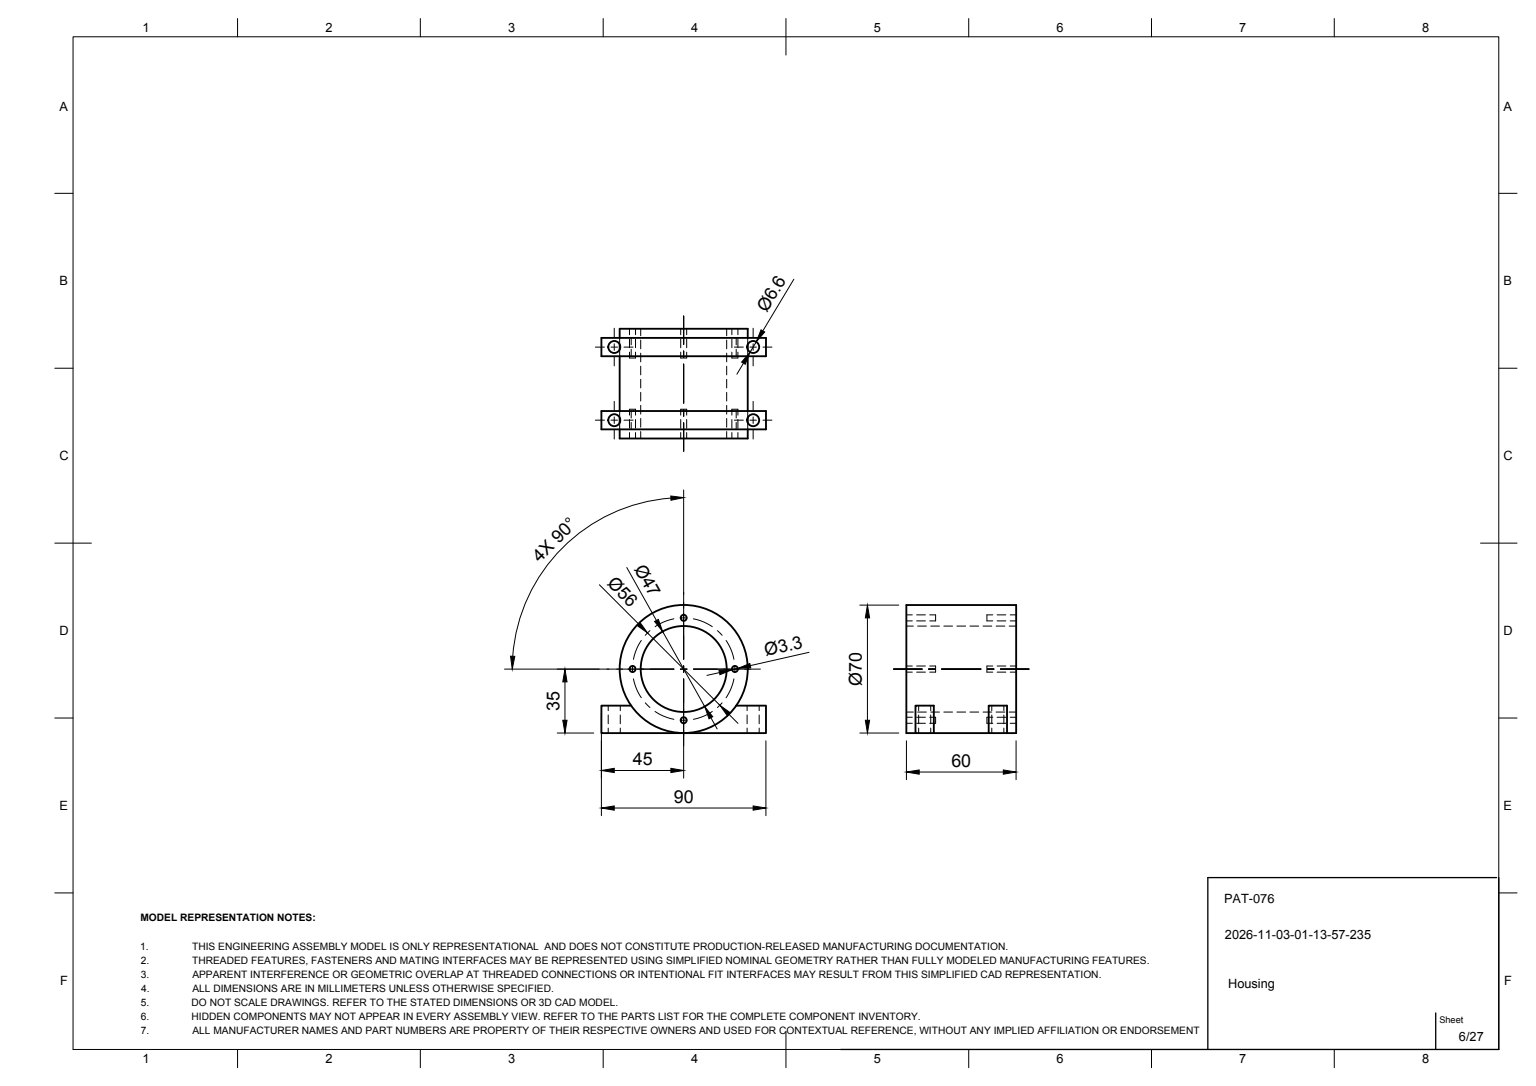
ISO-10303-21;
HEADER;
/* Generated by software containing ST-Developer
 * from STEP Tools, Inc. (www.steptools.com) 
 */

FILE_DESCRIPTION(
/* description */ ('Overhung pulley bearing cartridge'),
/* implementation_level */ '2;1');

FILE_NAME(
/* name */ 'Housing.step',
/* time_stamp */ '2026-10-28T03:22:33-07:00',
/* author */ (''),
/* organization */ (''),
/* preprocessor_version */ 'ST-DEVELOPER v20.2',
/* originating_system */ 'Autodesk Translation Framework v15.17.0.0',
/* authorisation */ '');

FILE_SCHEMA (('AUTOMOTIVE_DESIGN { 1 0 10303 214 3 1 1 }'));
ENDSEC;

DATA;
#10=MECHANICAL_DESIGN_GEOMETRIC_PRESENTATION_REPRESENTATION('',(#284),#10963);
#240=SHAPE_REPRESENTATION_RELATIONSHIP('SRR','None',#11060,#262);
#262=ADVANCED_BREP_SHAPE_REPRESENTATION('',(#314),#10940);
#284=STYLED_ITEM('',(#11232),#314);
#314=MANIFOLD_SOLID_BREP('Body1',#5651);
#349=FACE_BOUND('',#949,.T.);
#350=FACE_BOUND('',#951,.T.);
#351=FACE_BOUND('',#954,.T.);
#352=FACE_BOUND('',#955,.T.);
#353=FACE_BOUND('',#962,.T.);
#354=FACE_BOUND('',#964,.T.);
#355=FACE_BOUND('',#967,.T.);
#356=FACE_BOUND('',#968,.T.);
#357=FACE_BOUND('',#972,.T.);
#358=FACE_BOUND('',#973,.T.);
#359=FACE_BOUND('',#975,.T.);
#360=FACE_BOUND('',#976,.T.);
#361=FACE_BOUND('',#977,.T.);
#362=FACE_BOUND('',#978,.T.);
#363=FACE_BOUND('',#979,.T.);
#364=FACE_BOUND('',#981,.T.);
#365=FACE_BOUND('',#982,.T.);
#366=FACE_BOUND('',#983,.T.);
#367=FACE_BOUND('',#984,.T.);
#368=FACE_BOUND('',#985,.T.);
#440=PLANE('',#5950);
#441=PLANE('',#5954);
#442=PLANE('',#5958);
#443=PLANE('',#5962);
#444=PLANE('',#5966);
#445=PLANE('',#5970);
#446=PLANE('',#5974);
#447=PLANE('',#5978);
#448=PLANE('',#5991);
#449=PLANE('',#5993);
#450=PLANE('',#5995);
#451=PLANE('',#5997);
#452=PLANE('',#5999);
#453=PLANE('',#6000);
#454=PLANE('',#6001);
#455=PLANE('',#6002);
#456=PLANE('',#6003);
#457=PLANE('',#6004);
#458=PLANE('',#6006);
#459=PLANE('',#6008);
#460=PLANE('',#6010);
#461=PLANE('',#6012);
#462=PLANE('',#6013);
#463=PLANE('',#6014);
#464=PLANE('',#6015);
#465=PLANE('',#6016);
#466=PLANE('',#6023);
#467=PLANE('',#6024);
#587=FACE_OUTER_BOUND('',#924,.T.);
#588=FACE_OUTER_BOUND('',#925,.T.);
#589=FACE_OUTER_BOUND('',#926,.T.);
#590=FACE_OUTER_BOUND('',#927,.T.);
#591=FACE_OUTER_BOUND('',#928,.T.);
#592=FACE_OUTER_BOUND('',#929,.T.);
#593=FACE_OUTER_BOUND('',#930,.T.);
#594=FACE_OUTER_BOUND('',#931,.T.);
#595=FACE_OUTER_BOUND('',#932,.T.);
#596=FACE_OUTER_BOUND('',#933,.T.);
#597=FACE_OUTER_BOUND('',#934,.T.);
#598=FACE_OUTER_BOUND('',#935,.T.);
#599=FACE_OUTER_BOUND('',#936,.T.);
#600=FACE_OUTER_BOUND('',#937,.T.);
#601=FACE_OUTER_BOUND('',#938,.T.);
#602=FACE_OUTER_BOUND('',#939,.T.);
#603=FACE_OUTER_BOUND('',#940,.T.);
#604=FACE_OUTER_BOUND('',#941,.T.);
#605=FACE_OUTER_BOUND('',#942,.T.);
#606=FACE_OUTER_BOUND('',#943,.T.);
#607=FACE_OUTER_BOUND('',#944,.T.);
#608=FACE_OUTER_BOUND('',#945,.T.);
#609=FACE_OUTER_BOUND('',#946,.T.);
#610=FACE_OUTER_BOUND('',#947,.T.);
#611=FACE_OUTER_BOUND('',#948,.T.);
#612=FACE_OUTER_BOUND('',#950,.T.);
#613=FACE_OUTER_BOUND('',#952,.T.);
#614=FACE_OUTER_BOUND('',#953,.T.);
#615=FACE_OUTER_BOUND('',#956,.T.);
#616=FACE_OUTER_BOUND('',#957,.T.);
#617=FACE_OUTER_BOUND('',#958,.T.);
#618=FACE_OUTER_BOUND('',#959,.T.);
#619=FACE_OUTER_BOUND('',#960,.T.);
#620=FACE_OUTER_BOUND('',#961,.T.);
#621=FACE_OUTER_BOUND('',#963,.T.);
#622=FACE_OUTER_BOUND('',#965,.T.);
#623=FACE_OUTER_BOUND('',#966,.T.);
#624=FACE_OUTER_BOUND('',#969,.T.);
#625=FACE_OUTER_BOUND('',#970,.T.);
#626=FACE_OUTER_BOUND('',#971,.T.);
#627=FACE_OUTER_BOUND('',#974,.T.);
#628=FACE_OUTER_BOUND('',#980,.T.);
#924=EDGE_LOOP('',(#3701,#3702,#3703,#3704));
#925=EDGE_LOOP('',(#3705));
#926=EDGE_LOOP('',(#3706,#3707,#3708,#3709));
#927=EDGE_LOOP('',(#3710));
#928=EDGE_LOOP('',(#3711,#3712,#3713,#3714));
#929=EDGE_LOOP('',(#3715));
#930=EDGE_LOOP('',(#3716,#3717,#3718,#3719));
#931=EDGE_LOOP('',(#3720));
#932=EDGE_LOOP('',(#3721,#3722,#3723,#3724));
#933=EDGE_LOOP('',(#3725));
#934=EDGE_LOOP('',(#3726,#3727,#3728,#3729));
#935=EDGE_LOOP('',(#3730));
#936=EDGE_LOOP('',(#3731,#3732,#3733,#3734));
#937=EDGE_LOOP('',(#3735));
#938=EDGE_LOOP('',(#3736,#3737,#3738,#3739));
#939=EDGE_LOOP('',(#3740));
#940=EDGE_LOOP('',(#3741,#3742,#3743,#3744));
#941=EDGE_LOOP('',(#3745,#3746,#3747,#3748));
#942=EDGE_LOOP('',(#3749,#3750,#3751,#3752));
#943=EDGE_LOOP('',(#3753,#3754,#3755,#3756));
#944=EDGE_LOOP('',(#3757,#3758,#3759,#3760));
#945=EDGE_LOOP('',(#3761,#3762,#3763,#3764));
#946=EDGE_LOOP('',(#3765,#3766,#3767,#3768));
#947=EDGE_LOOP('',(#3769,#3770,#3771,#3772));
#948=EDGE_LOOP('',(#3773,#3774,#3775,#3776));
#949=EDGE_LOOP('',(#3777));
#950=EDGE_LOOP('',(#3778,#3779,#3780,#3781));
#951=EDGE_LOOP('',(#3782));
#952=EDGE_LOOP('',(#3783,#3784,#3785,#3786));
#953=EDGE_LOOP('',(#3787,#3788,#3789,#3790,#3791,#3792));
#954=EDGE_LOOP('',(#3793));
#955=EDGE_LOOP('',(#3794));
#956=EDGE_LOOP('',(#3795,#3796,#3797,#3798));
#957=EDGE_LOOP('',(#3799,#3800,#3801,#3802));
#958=EDGE_LOOP('',(#3803,#3804,#3805,#3806));
#959=EDGE_LOOP('',(#3807,#3808,#3809,#3810));
#960=EDGE_LOOP('',(#3811,#3812,#3813,#3814));
#961=EDGE_LOOP('',(#3815,#3816,#3817,#3818));
#962=EDGE_LOOP('',(#3819));
#963=EDGE_LOOP('',(#3820,#3821,#3822,#3823));
#964=EDGE_LOOP('',(#3824));
#965=EDGE_LOOP('',(#3825,#3826,#3827,#3828));
#966=EDGE_LOOP('',(#3829,#3830,#3831,#3832,#3833,#3834));
#967=EDGE_LOOP('',(#3835));
#968=EDGE_LOOP('',(#3836));
#969=EDGE_LOOP('',(#3837,#3838,#3839,#3840));
#970=EDGE_LOOP('',(#3841,#3842,#3843,#3844));
#971=EDGE_LOOP('',(#3845,#3846,#3847,#3848));
#972=EDGE_LOOP('',(#3849,#3850,#3851,#3852,#3853,#3854));
#973=EDGE_LOOP('',(#3855,#3856,#3857,#3858,#3859,#3860));
#974=EDGE_LOOP('',(#3861));
#975=EDGE_LOOP('',(#3862));
#976=EDGE_LOOP('',(#3863));
#977=EDGE_LOOP('',(#3864));
#978=EDGE_LOOP('',(#3865));
#979=EDGE_LOOP('',(#3866));
#980=EDGE_LOOP('',(#3867));
#981=EDGE_LOOP('',(#3868));
#982=EDGE_LOOP('',(#3869));
#983=EDGE_LOOP('',(#3870));
#984=EDGE_LOOP('',(#3871));
#985=EDGE_LOOP('',(#3872));
#1344=LINE('',#8614,#1686);
#1345=LINE('',#8621,#1687);
#1346=LINE('',#8628,#1688);
#1347=LINE('',#8635,#1689);
#1348=LINE('',#8642,#1690);
#1349=LINE('',#8649,#1691);
#1350=LINE('',#8656,#1692);
#1351=LINE('',#8663,#1693);
#1352=LINE('',#8670,#1694);
#1353=LINE('',#8676,#1695);
#1354=LINE('',#8682,#1696);
#1355=LINE('',#8688,#1697);
#1356=LINE('',#8695,#1698);
#1357=LINE('',#8697,#1699);
#1358=LINE('',#8698,#1700);
#1359=LINE('',#8703,#1701);
#1360=LINE('',#8705,#1702);
#1361=LINE('',#8706,#1703);
#1362=LINE('',#8712,#1704);
#1363=LINE('',#8714,#1705);
#1364=LINE('',#8715,#1706);
#1365=LINE('',#8720,#1707);
#1366=LINE('',#8722,#1708);
#1367=LINE('',#8723,#1709);
#1368=LINE('',#8725,#1710);
#1369=LINE('',#8726,#1711);
#1370=LINE('',#8728,#1712);
#1371=LINE('',#8729,#1713);
#1372=LINE('',#8731,#1714);
#1373=LINE('',#8733,#1715);
#1374=LINE('',#8740,#1716);
#1375=LINE('',#8742,#1717);
#1376=LINE('',#8743,#1718);
#1377=LINE('',#8748,#1719);
#1378=LINE('',#8750,#1720);
#1379=LINE('',#8751,#1721);
#1380=LINE('',#8757,#1722);
#1381=LINE('',#8759,#1723);
#1382=LINE('',#8760,#1724);
#1383=LINE('',#8765,#1725);
#1384=LINE('',#8767,#1726);
#1385=LINE('',#8768,#1727);
#1386=LINE('',#8770,#1728);
#1387=LINE('',#8771,#1729);
#1388=LINE('',#8773,#1730);
#1389=LINE('',#8774,#1731);
#1390=LINE('',#8776,#1732);
#1391=LINE('',#8778,#1733);
#1392=LINE('',#8784,#1734);
#1393=LINE('',#8790,#1735);
#1686=VECTOR('',#6752,0.165);
#1687=VECTOR('',#6761,0.165);
#1688=VECTOR('',#6770,0.165);
#1689=VECTOR('',#6779,0.165);
#1690=VECTOR('',#6788,0.165);
#1691=VECTOR('',#6797,0.165);
#1692=VECTOR('',#6806,0.165);
#1693=VECTOR('',#6815,0.165);
#1694=VECTOR('',#6824,0.33);
#1695=VECTOR('',#6831,0.33);
#1696=VECTOR('',#6838,0.33);
#1697=VECTOR('',#6845,0.33);
#1698=VECTOR('',#6852,1.);
#1699=VECTOR('',#6853,1.);
#1700=VECTOR('',#6854,1.);
#1701=VECTOR('',#6859,1.);
#1702=VECTOR('',#6860,1.);
#1703=VECTOR('',#6861,1.);
#1704=VECTOR('',#6866,1.);
#1705=VECTOR('',#6867,1.);
#1706=VECTOR('',#6868,1.);
#1707=VECTOR('',#6873,1.);
#1708=VECTOR('',#6874,1.);
#1709=VECTOR('',#6875,1.);
#1710=VECTOR('',#6878,1.);
#1711=VECTOR('',#6879,1.);
#1712=VECTOR('',#6882,1.);
#1713=VECTOR('',#6883,1.);
#1714=VECTOR('',#6886,1.);
#1715=VECTOR('',#6889,1.);
#1716=VECTOR('',#6896,1.);
#1717=VECTOR('',#6897,1.);
#1718=VECTOR('',#6898,1.);
#1719=VECTOR('',#6903,1.);
#1720=VECTOR('',#6904,1.);
#1721=VECTOR('',#6905,1.);
#1722=VECTOR('',#6910,1.);
#1723=VECTOR('',#6911,1.);
#1724=VECTOR('',#6912,1.);
#1725=VECTOR('',#6917,1.);
#1726=VECTOR('',#6918,1.);
#1727=VECTOR('',#6919,1.);
#1728=VECTOR('',#6922,1.);
#1729=VECTOR('',#6923,1.);
#1730=VECTOR('',#6926,1.);
#1731=VECTOR('',#6927,1.);
#1732=VECTOR('',#6930,1.);
#1733=VECTOR('',#6933,1.);
#1734=VECTOR('',#6940,2.35);
#1735=VECTOR('',#6947,3.5);
#2020=CIRCLE('',#5948,0.165);
#2021=CIRCLE('',#5949,0.165);
#2022=CIRCLE('',#5952,0.165);
#2023=CIRCLE('',#5953,0.165);
#2024=CIRCLE('',#5956,0.165);
#2025=CIRCLE('',#5957,0.165);
#2026=CIRCLE('',#5960,0.165);
#2027=CIRCLE('',#5961,0.165);
#2028=CIRCLE('',#5964,0.165);
#2029=CIRCLE('',#5965,0.165);
#2030=CIRCLE('',#5968,0.165);
#2031=CIRCLE('',#5969,0.165);
#2032=CIRCLE('',#5972,0.165);
#2033=CIRCLE('',#5973,0.165);
#2034=CIRCLE('',#5976,0.165);
#2035=CIRCLE('',#5977,0.165);
#2036=CIRCLE('',#5980,0.33);
#2037=CIRCLE('',#5981,0.33);
#2038=CIRCLE('',#5983,0.33);
#2039=CIRCLE('',#5984,0.33);
#2040=CIRCLE('',#5986,0.33);
#2041=CIRCLE('',#5987,0.33);
#2042=CIRCLE('',#5989,0.33);
#2043=CIRCLE('',#5990,0.33);
#2044=CIRCLE('',#5992,3.5);
#2045=CIRCLE('',#5994,3.5);
#2046=CIRCLE('',#5996,3.5);
#2047=CIRCLE('',#5998,3.5);
#2048=CIRCLE('',#6005,3.5);
#2049=CIRCLE('',#6007,3.5);
#2050=CIRCLE('',#6009,3.5);
#2051=CIRCLE('',#6011,3.5);
#2052=CIRCLE('',#6018,2.35);
#2053=CIRCLE('',#6019,2.35);
#2054=CIRCLE('',#6021,3.5);
#2055=CIRCLE('',#6022,3.5);
#2399=VERTEX_POINT('',#8611);
#2400=VERTEX_POINT('',#8613);
#2401=VERTEX_POINT('',#8618);
#2402=VERTEX_POINT('',#8620);
#2403=VERTEX_POINT('',#8625);
#2404=VERTEX_POINT('',#8627);
#2405=VERTEX_POINT('',#8632);
#2406=VERTEX_POINT('',#8634);
#2407=VERTEX_POINT('',#8639);
#2408=VERTEX_POINT('',#8641);
#2409=VERTEX_POINT('',#8646);
#2410=VERTEX_POINT('',#8648);
#2411=VERTEX_POINT('',#8653);
#2412=VERTEX_POINT('',#8655);
#2413=VERTEX_POINT('',#8660);
#2414=VERTEX_POINT('',#8662);
#2415=VERTEX_POINT('',#8667);
#2416=VERTEX_POINT('',#8669);
#2417=VERTEX_POINT('',#8673);
#2418=VERTEX_POINT('',#8675);
#2419=VERTEX_POINT('',#8679);
#2420=VERTEX_POINT('',#8681);
#2421=VERTEX_POINT('',#8685);
#2422=VERTEX_POINT('',#8687);
#2423=VERTEX_POINT('',#8691);
#2424=VERTEX_POINT('',#8692);
#2425=VERTEX_POINT('',#8694);
#2426=VERTEX_POINT('',#8696);
#2427=VERTEX_POINT('',#8700);
#2428=VERTEX_POINT('',#8702);
#2429=VERTEX_POINT('',#8704);
#2430=VERTEX_POINT('',#8708);
#2431=VERTEX_POINT('',#8709);
#2432=VERTEX_POINT('',#8711);
#2433=VERTEX_POINT('',#8713);
#2434=VERTEX_POINT('',#8717);
#2435=VERTEX_POINT('',#8719);
#2436=VERTEX_POINT('',#8721);
#2437=VERTEX_POINT('',#8736);
#2438=VERTEX_POINT('',#8737);
#2439=VERTEX_POINT('',#8739);
#2440=VERTEX_POINT('',#8741);
#2441=VERTEX_POINT('',#8745);
#2442=VERTEX_POINT('',#8747);
#2443=VERTEX_POINT('',#8749);
#2444=VERTEX_POINT('',#8753);
#2445=VERTEX_POINT('',#8754);
#2446=VERTEX_POINT('',#8756);
#2447=VERTEX_POINT('',#8758);
#2448=VERTEX_POINT('',#8762);
#2449=VERTEX_POINT('',#8764);
#2450=VERTEX_POINT('',#8766);
#2451=VERTEX_POINT('',#8781);
#2452=VERTEX_POINT('',#8783);
#2453=VERTEX_POINT('',#8787);
#2454=VERTEX_POINT('',#8789);
#2920=EDGE_CURVE('',#2399,#2399,#2020,.T.);
#2921=EDGE_CURVE('',#2399,#2400,#1344,.T.);
#2922=EDGE_CURVE('',#2400,#2400,#2021,.T.);
#2923=EDGE_CURVE('',#2401,#2401,#2022,.T.);
#2924=EDGE_CURVE('',#2401,#2402,#1345,.T.);
#2925=EDGE_CURVE('',#2402,#2402,#2023,.T.);
#2926=EDGE_CURVE('',#2403,#2403,#2024,.T.);
#2927=EDGE_CURVE('',#2403,#2404,#1346,.T.);
#2928=EDGE_CURVE('',#2404,#2404,#2025,.T.);
#2929=EDGE_CURVE('',#2405,#2405,#2026,.T.);
#2930=EDGE_CURVE('',#2405,#2406,#1347,.T.);
#2931=EDGE_CURVE('',#2406,#2406,#2027,.T.);
#2932=EDGE_CURVE('',#2407,#2407,#2028,.T.);
#2933=EDGE_CURVE('',#2407,#2408,#1348,.T.);
#2934=EDGE_CURVE('',#2408,#2408,#2029,.T.);
#2935=EDGE_CURVE('',#2409,#2409,#2030,.T.);
#2936=EDGE_CURVE('',#2409,#2410,#1349,.T.);
#2937=EDGE_CURVE('',#2410,#2410,#2031,.T.);
#2938=EDGE_CURVE('',#2411,#2411,#2032,.T.);
#2939=EDGE_CURVE('',#2411,#2412,#1350,.T.);
#2940=EDGE_CURVE('',#2412,#2412,#2033,.T.);
#2941=EDGE_CURVE('',#2413,#2413,#2034,.T.);
#2942=EDGE_CURVE('',#2413,#2414,#1351,.T.);
#2943=EDGE_CURVE('',#2414,#2414,#2035,.T.);
#2944=EDGE_CURVE('',#2415,#2415,#2036,.T.);
#2945=EDGE_CURVE('',#2415,#2416,#1352,.T.);
#2946=EDGE_CURVE('',#2416,#2416,#2037,.T.);
#2947=EDGE_CURVE('',#2417,#2417,#2038,.T.);
#2948=EDGE_CURVE('',#2417,#2418,#1353,.T.);
#2949=EDGE_CURVE('',#2418,#2418,#2039,.T.);
#2950=EDGE_CURVE('',#2419,#2419,#2040,.T.);
#2951=EDGE_CURVE('',#2419,#2420,#1354,.T.);
#2952=EDGE_CURVE('',#2420,#2420,#2041,.T.);
#2953=EDGE_CURVE('',#2421,#2421,#2042,.T.);
#2954=EDGE_CURVE('',#2421,#2422,#1355,.T.);
#2955=EDGE_CURVE('',#2422,#2422,#2043,.T.);
#2956=EDGE_CURVE('',#2423,#2424,#2044,.T.);
#2957=EDGE_CURVE('',#2423,#2425,#1356,.T.);
#2958=EDGE_CURVE('',#2425,#2426,#1357,.T.);
#2959=EDGE_CURVE('',#2426,#2424,#1358,.T.);
#2960=EDGE_CURVE('',#2424,#2427,#2045,.T.);
#2961=EDGE_CURVE('',#2424,#2428,#1359,.T.);
#2962=EDGE_CURVE('',#2428,#2429,#1360,.T.);
#2963=EDGE_CURVE('',#2429,#2427,#1361,.T.);
#2964=EDGE_CURVE('',#2430,#2431,#2046,.T.);
#2965=EDGE_CURVE('',#2430,#2432,#1362,.T.);
#2966=EDGE_CURVE('',#2432,#2433,#1363,.T.);
#2967=EDGE_CURVE('',#2433,#2431,#1364,.T.);
#2968=EDGE_CURVE('',#2434,#2430,#2047,.T.);
#2969=EDGE_CURVE('',#2434,#2435,#1365,.T.);
#2970=EDGE_CURVE('',#2435,#2436,#1366,.T.);
#2971=EDGE_CURVE('',#2436,#2430,#1367,.T.);
#2972=EDGE_CURVE('',#2431,#2423,#1368,.T.);
#2973=EDGE_CURVE('',#2433,#2425,#1369,.T.);
#2974=EDGE_CURVE('',#2427,#2434,#1370,.T.);
#2975=EDGE_CURVE('',#2435,#2429,#1371,.T.);
#2976=EDGE_CURVE('',#2436,#2428,#1372,.T.);
#2977=EDGE_CURVE('',#2432,#2426,#1373,.T.);
#2978=EDGE_CURVE('',#2437,#2438,#2048,.T.);
#2979=EDGE_CURVE('',#2437,#2439,#1374,.T.);
#2980=EDGE_CURVE('',#2439,#2440,#1375,.T.);
#2981=EDGE_CURVE('',#2440,#2438,#1376,.T.);
#2982=EDGE_CURVE('',#2438,#2441,#2049,.T.);
#2983=EDGE_CURVE('',#2438,#2442,#1377,.T.);
#2984=EDGE_CURVE('',#2442,#2443,#1378,.T.);
#2985=EDGE_CURVE('',#2443,#2441,#1379,.T.);
#2986=EDGE_CURVE('',#2444,#2445,#2050,.T.);
#2987=EDGE_CURVE('',#2444,#2446,#1380,.T.);
#2988=EDGE_CURVE('',#2446,#2447,#1381,.T.);
#2989=EDGE_CURVE('',#2447,#2445,#1382,.T.);
#2990=EDGE_CURVE('',#2448,#2444,#2051,.T.);
#2991=EDGE_CURVE('',#2448,#2449,#1383,.T.);
#2992=EDGE_CURVE('',#2449,#2450,#1384,.T.);
#2993=EDGE_CURVE('',#2450,#2444,#1385,.T.);
#2994=EDGE_CURVE('',#2445,#2437,#1386,.T.);
#2995=EDGE_CURVE('',#2447,#2439,#1387,.T.);
#2996=EDGE_CURVE('',#2441,#2448,#1388,.T.);
#2997=EDGE_CURVE('',#2449,#2443,#1389,.T.);
#2998=EDGE_CURVE('',#2450,#2442,#1390,.T.);
#2999=EDGE_CURVE('',#2446,#2440,#1391,.T.);
#3000=EDGE_CURVE('',#2451,#2451,#2052,.T.);
#3001=EDGE_CURVE('',#2451,#2452,#1392,.T.);
#3002=EDGE_CURVE('',#2452,#2452,#2053,.T.);
#3003=EDGE_CURVE('',#2453,#2453,#2054,.T.);
#3004=EDGE_CURVE('',#2453,#2454,#1393,.T.);
#3005=EDGE_CURVE('',#2454,#2454,#2055,.T.);
#3701=ORIENTED_EDGE('',*,*,#2920,.F.);
#3702=ORIENTED_EDGE('',*,*,#2921,.T.);
#3703=ORIENTED_EDGE('',*,*,#2922,.F.);
#3704=ORIENTED_EDGE('',*,*,#2921,.F.);
#3705=ORIENTED_EDGE('',*,*,#2920,.T.);
#3706=ORIENTED_EDGE('',*,*,#2923,.F.);
#3707=ORIENTED_EDGE('',*,*,#2924,.T.);
#3708=ORIENTED_EDGE('',*,*,#2925,.F.);
#3709=ORIENTED_EDGE('',*,*,#2924,.F.);
#3710=ORIENTED_EDGE('',*,*,#2923,.T.);
#3711=ORIENTED_EDGE('',*,*,#2926,.F.);
#3712=ORIENTED_EDGE('',*,*,#2927,.T.);
#3713=ORIENTED_EDGE('',*,*,#2928,.F.);
#3714=ORIENTED_EDGE('',*,*,#2927,.F.);
#3715=ORIENTED_EDGE('',*,*,#2926,.T.);
#3716=ORIENTED_EDGE('',*,*,#2929,.F.);
#3717=ORIENTED_EDGE('',*,*,#2930,.T.);
#3718=ORIENTED_EDGE('',*,*,#2931,.F.);
#3719=ORIENTED_EDGE('',*,*,#2930,.F.);
#3720=ORIENTED_EDGE('',*,*,#2929,.T.);
#3721=ORIENTED_EDGE('',*,*,#2932,.F.);
#3722=ORIENTED_EDGE('',*,*,#2933,.T.);
#3723=ORIENTED_EDGE('',*,*,#2934,.T.);
#3724=ORIENTED_EDGE('',*,*,#2933,.F.);
#3725=ORIENTED_EDGE('',*,*,#2934,.F.);
#3726=ORIENTED_EDGE('',*,*,#2935,.F.);
#3727=ORIENTED_EDGE('',*,*,#2936,.T.);
#3728=ORIENTED_EDGE('',*,*,#2937,.T.);
#3729=ORIENTED_EDGE('',*,*,#2936,.F.);
#3730=ORIENTED_EDGE('',*,*,#2937,.F.);
#3731=ORIENTED_EDGE('',*,*,#2938,.F.);
#3732=ORIENTED_EDGE('',*,*,#2939,.T.);
#3733=ORIENTED_EDGE('',*,*,#2940,.T.);
#3734=ORIENTED_EDGE('',*,*,#2939,.F.);
#3735=ORIENTED_EDGE('',*,*,#2940,.F.);
#3736=ORIENTED_EDGE('',*,*,#2941,.F.);
#3737=ORIENTED_EDGE('',*,*,#2942,.T.);
#3738=ORIENTED_EDGE('',*,*,#2943,.T.);
#3739=ORIENTED_EDGE('',*,*,#2942,.F.);
#3740=ORIENTED_EDGE('',*,*,#2943,.F.);
#3741=ORIENTED_EDGE('',*,*,#2944,.F.);
#3742=ORIENTED_EDGE('',*,*,#2945,.T.);
#3743=ORIENTED_EDGE('',*,*,#2946,.F.);
#3744=ORIENTED_EDGE('',*,*,#2945,.F.);
#3745=ORIENTED_EDGE('',*,*,#2947,.F.);
#3746=ORIENTED_EDGE('',*,*,#2948,.T.);
#3747=ORIENTED_EDGE('',*,*,#2949,.F.);
#3748=ORIENTED_EDGE('',*,*,#2948,.F.);
#3749=ORIENTED_EDGE('',*,*,#2950,.F.);
#3750=ORIENTED_EDGE('',*,*,#2951,.T.);
#3751=ORIENTED_EDGE('',*,*,#2952,.F.);
#3752=ORIENTED_EDGE('',*,*,#2951,.F.);
#3753=ORIENTED_EDGE('',*,*,#2953,.F.);
#3754=ORIENTED_EDGE('',*,*,#2954,.T.);
#3755=ORIENTED_EDGE('',*,*,#2955,.F.);
#3756=ORIENTED_EDGE('',*,*,#2954,.F.);
#3757=ORIENTED_EDGE('',*,*,#2956,.F.);
#3758=ORIENTED_EDGE('',*,*,#2957,.T.);
#3759=ORIENTED_EDGE('',*,*,#2958,.T.);
#3760=ORIENTED_EDGE('',*,*,#2959,.T.);
#3761=ORIENTED_EDGE('',*,*,#2960,.F.);
#3762=ORIENTED_EDGE('',*,*,#2961,.T.);
#3763=ORIENTED_EDGE('',*,*,#2962,.T.);
#3764=ORIENTED_EDGE('',*,*,#2963,.T.);
#3765=ORIENTED_EDGE('',*,*,#2964,.F.);
#3766=ORIENTED_EDGE('',*,*,#2965,.T.);
#3767=ORIENTED_EDGE('',*,*,#2966,.T.);
#3768=ORIENTED_EDGE('',*,*,#2967,.T.);
#3769=ORIENTED_EDGE('',*,*,#2968,.F.);
#3770=ORIENTED_EDGE('',*,*,#2969,.T.);
#3771=ORIENTED_EDGE('',*,*,#2970,.T.);
#3772=ORIENTED_EDGE('',*,*,#2971,.T.);
#3773=ORIENTED_EDGE('',*,*,#2972,.F.);
#3774=ORIENTED_EDGE('',*,*,#2967,.F.);
#3775=ORIENTED_EDGE('',*,*,#2973,.T.);
#3776=ORIENTED_EDGE('',*,*,#2957,.F.);
#3777=ORIENTED_EDGE('',*,*,#2955,.T.);
#3778=ORIENTED_EDGE('',*,*,#2974,.F.);
#3779=ORIENTED_EDGE('',*,*,#2963,.F.);
#3780=ORIENTED_EDGE('',*,*,#2975,.F.);
#3781=ORIENTED_EDGE('',*,*,#2969,.F.);
#3782=ORIENTED_EDGE('',*,*,#2949,.T.);
#3783=ORIENTED_EDGE('',*,*,#2970,.F.);
#3784=ORIENTED_EDGE('',*,*,#2975,.T.);
#3785=ORIENTED_EDGE('',*,*,#2962,.F.);
#3786=ORIENTED_EDGE('',*,*,#2976,.F.);
#3787=ORIENTED_EDGE('',*,*,#2959,.F.);
#3788=ORIENTED_EDGE('',*,*,#2977,.F.);
#3789=ORIENTED_EDGE('',*,*,#2965,.F.);
#3790=ORIENTED_EDGE('',*,*,#2971,.F.);
#3791=ORIENTED_EDGE('',*,*,#2976,.T.);
#3792=ORIENTED_EDGE('',*,*,#2961,.F.);
#3793=ORIENTED_EDGE('',*,*,#2947,.T.);
#3794=ORIENTED_EDGE('',*,*,#2953,.T.);
#3795=ORIENTED_EDGE('',*,*,#2966,.F.);
#3796=ORIENTED_EDGE('',*,*,#2977,.T.);
#3797=ORIENTED_EDGE('',*,*,#2958,.F.);
#3798=ORIENTED_EDGE('',*,*,#2973,.F.);
#3799=ORIENTED_EDGE('',*,*,#2978,.F.);
#3800=ORIENTED_EDGE('',*,*,#2979,.T.);
#3801=ORIENTED_EDGE('',*,*,#2980,.T.);
#3802=ORIENTED_EDGE('',*,*,#2981,.T.);
#3803=ORIENTED_EDGE('',*,*,#2982,.F.);
#3804=ORIENTED_EDGE('',*,*,#2983,.T.);
#3805=ORIENTED_EDGE('',*,*,#2984,.T.);
#3806=ORIENTED_EDGE('',*,*,#2985,.T.);
#3807=ORIENTED_EDGE('',*,*,#2986,.F.);
#3808=ORIENTED_EDGE('',*,*,#2987,.T.);
#3809=ORIENTED_EDGE('',*,*,#2988,.T.);
#3810=ORIENTED_EDGE('',*,*,#2989,.T.);
#3811=ORIENTED_EDGE('',*,*,#2990,.F.);
#3812=ORIENTED_EDGE('',*,*,#2991,.T.);
#3813=ORIENTED_EDGE('',*,*,#2992,.T.);
#3814=ORIENTED_EDGE('',*,*,#2993,.T.);
#3815=ORIENTED_EDGE('',*,*,#2994,.F.);
#3816=ORIENTED_EDGE('',*,*,#2989,.F.);
#3817=ORIENTED_EDGE('',*,*,#2995,.T.);
#3818=ORIENTED_EDGE('',*,*,#2979,.F.);
#3819=ORIENTED_EDGE('',*,*,#2946,.T.);
#3820=ORIENTED_EDGE('',*,*,#2996,.F.);
#3821=ORIENTED_EDGE('',*,*,#2985,.F.);
#3822=ORIENTED_EDGE('',*,*,#2997,.F.);
#3823=ORIENTED_EDGE('',*,*,#2991,.F.);
#3824=ORIENTED_EDGE('',*,*,#2952,.T.);
#3825=ORIENTED_EDGE('',*,*,#2992,.F.);
#3826=ORIENTED_EDGE('',*,*,#2997,.T.);
#3827=ORIENTED_EDGE('',*,*,#2984,.F.);
#3828=ORIENTED_EDGE('',*,*,#2998,.F.);
#3829=ORIENTED_EDGE('',*,*,#2981,.F.);
#3830=ORIENTED_EDGE('',*,*,#2999,.F.);
#3831=ORIENTED_EDGE('',*,*,#2987,.F.);
#3832=ORIENTED_EDGE('',*,*,#2993,.F.);
#3833=ORIENTED_EDGE('',*,*,#2998,.T.);
#3834=ORIENTED_EDGE('',*,*,#2983,.F.);
#3835=ORIENTED_EDGE('',*,*,#2944,.T.);
#3836=ORIENTED_EDGE('',*,*,#2950,.T.);
#3837=ORIENTED_EDGE('',*,*,#2988,.F.);
#3838=ORIENTED_EDGE('',*,*,#2999,.T.);
#3839=ORIENTED_EDGE('',*,*,#2980,.F.);
#3840=ORIENTED_EDGE('',*,*,#2995,.F.);
#3841=ORIENTED_EDGE('',*,*,#3000,.F.);
#3842=ORIENTED_EDGE('',*,*,#3001,.T.);
#3843=ORIENTED_EDGE('',*,*,#3002,.T.);
#3844=ORIENTED_EDGE('',*,*,#3001,.F.);
#3845=ORIENTED_EDGE('',*,*,#3003,.F.);
#3846=ORIENTED_EDGE('',*,*,#3004,.T.);
#3847=ORIENTED_EDGE('',*,*,#3005,.T.);
#3848=ORIENTED_EDGE('',*,*,#3004,.F.);
#3849=ORIENTED_EDGE('',*,*,#2972,.T.);
#3850=ORIENTED_EDGE('',*,*,#2956,.T.);
#3851=ORIENTED_EDGE('',*,*,#2960,.T.);
#3852=ORIENTED_EDGE('',*,*,#2974,.T.);
#3853=ORIENTED_EDGE('',*,*,#2968,.T.);
#3854=ORIENTED_EDGE('',*,*,#2964,.T.);
#3855=ORIENTED_EDGE('',*,*,#2994,.T.);
#3856=ORIENTED_EDGE('',*,*,#2978,.T.);
#3857=ORIENTED_EDGE('',*,*,#2982,.T.);
#3858=ORIENTED_EDGE('',*,*,#2996,.T.);
#3859=ORIENTED_EDGE('',*,*,#2990,.T.);
#3860=ORIENTED_EDGE('',*,*,#2986,.T.);
#3861=ORIENTED_EDGE('',*,*,#3003,.T.);
#3862=ORIENTED_EDGE('',*,*,#3000,.T.);
#3863=ORIENTED_EDGE('',*,*,#2931,.T.);
#3864=ORIENTED_EDGE('',*,*,#2928,.T.);
#3865=ORIENTED_EDGE('',*,*,#2925,.T.);
#3866=ORIENTED_EDGE('',*,*,#2922,.T.);
#3867=ORIENTED_EDGE('',*,*,#3005,.F.);
#3868=ORIENTED_EDGE('',*,*,#3002,.F.);
#3869=ORIENTED_EDGE('',*,*,#2941,.T.);
#3870=ORIENTED_EDGE('',*,*,#2938,.T.);
#3871=ORIENTED_EDGE('',*,*,#2935,.T.);
#3872=ORIENTED_EDGE('',*,*,#2932,.T.);
#5171=CYLINDRICAL_SURFACE('',#5947,0.165);
#5172=CYLINDRICAL_SURFACE('',#5951,0.165);
#5173=CYLINDRICAL_SURFACE('',#5955,0.165);
#5174=CYLINDRICAL_SURFACE('',#5959,0.165);
#5175=CYLINDRICAL_SURFACE('',#5963,0.165);
#5176=CYLINDRICAL_SURFACE('',#5967,0.165);
#5177=CYLINDRICAL_SURFACE('',#5971,0.165);
#5178=CYLINDRICAL_SURFACE('',#5975,0.165);
#5179=CYLINDRICAL_SURFACE('',#5979,0.33);
#5180=CYLINDRICAL_SURFACE('',#5982,0.33);
#5181=CYLINDRICAL_SURFACE('',#5985,0.33);
#5182=CYLINDRICAL_SURFACE('',#5988,0.33);
#5183=CYLINDRICAL_SURFACE('',#6017,2.35);
#5184=CYLINDRICAL_SURFACE('',#6020,3.5);
#5331=ADVANCED_FACE('',(#587),#5171,.F.);
#5332=ADVANCED_FACE('',(#588),#440,.T.);
#5333=ADVANCED_FACE('',(#589),#5172,.F.);
#5334=ADVANCED_FACE('',(#590),#441,.T.);
#5335=ADVANCED_FACE('',(#591),#5173,.F.);
#5336=ADVANCED_FACE('',(#592),#442,.T.);
#5337=ADVANCED_FACE('',(#593),#5174,.F.);
#5338=ADVANCED_FACE('',(#594),#443,.T.);
#5339=ADVANCED_FACE('',(#595),#5175,.F.);
#5340=ADVANCED_FACE('',(#596),#444,.F.);
#5341=ADVANCED_FACE('',(#597),#5176,.F.);
#5342=ADVANCED_FACE('',(#598),#445,.F.);
#5343=ADVANCED_FACE('',(#599),#5177,.F.);
#5344=ADVANCED_FACE('',(#600),#446,.F.);
#5345=ADVANCED_FACE('',(#601),#5178,.F.);
#5346=ADVANCED_FACE('',(#602),#447,.F.);
#5347=ADVANCED_FACE('',(#603),#5179,.F.);
#5348=ADVANCED_FACE('',(#604),#5180,.F.);
#5349=ADVANCED_FACE('',(#605),#5181,.F.);
#5350=ADVANCED_FACE('',(#606),#5182,.F.);
#5351=ADVANCED_FACE('',(#607),#448,.T.);
#5352=ADVANCED_FACE('',(#608),#449,.T.);
#5353=ADVANCED_FACE('',(#609),#450,.F.);
#5354=ADVANCED_FACE('',(#610),#451,.F.);
#5355=ADVANCED_FACE('',(#611,#349),#452,.T.);
#5356=ADVANCED_FACE('',(#612,#350),#453,.T.);
#5357=ADVANCED_FACE('',(#613),#454,.T.);
#5358=ADVANCED_FACE('',(#614,#351,#352),#455,.T.);
#5359=ADVANCED_FACE('',(#615),#456,.T.);
#5360=ADVANCED_FACE('',(#616),#457,.T.);
#5361=ADVANCED_FACE('',(#617),#458,.T.);
#5362=ADVANCED_FACE('',(#618),#459,.F.);
#5363=ADVANCED_FACE('',(#619),#460,.F.);
#5364=ADVANCED_FACE('',(#620,#353),#461,.T.);
#5365=ADVANCED_FACE('',(#621,#354),#462,.T.);
#5366=ADVANCED_FACE('',(#622),#463,.T.);
#5367=ADVANCED_FACE('',(#623,#355,#356),#464,.T.);
#5368=ADVANCED_FACE('',(#624),#465,.T.);
#5369=ADVANCED_FACE('',(#625),#5183,.F.);
#5370=ADVANCED_FACE('',(#626,#357,#358),#5184,.T.);
#5371=ADVANCED_FACE('',(#627,#359,#360,#361,#362,#363),#466,.T.);
#5372=ADVANCED_FACE('',(#628,#364,#365,#366,#367,#368),#467,.F.);
#5651=CLOSED_SHELL('',(#5331,#5332,#5333,#5334,#5335,#5336,#5337,#5338,
#5339,#5340,#5341,#5342,#5343,#5344,#5345,#5346,#5347,#5348,#5349,#5350,
#5351,#5352,#5353,#5354,#5355,#5356,#5357,#5358,#5359,#5360,#5361,#5362,
#5363,#5364,#5365,#5366,#5367,#5368,#5369,#5370,#5371,#5372));
#5946=AXIS2_PLACEMENT_3D('',#8609,#6746,#6747);
#5947=AXIS2_PLACEMENT_3D('',#8610,#6748,#6749);
#5948=AXIS2_PLACEMENT_3D('',#8612,#6750,#6751);
#5949=AXIS2_PLACEMENT_3D('',#8615,#6753,#6754);
#5950=AXIS2_PLACEMENT_3D('',#8616,#6755,#6756);
#5951=AXIS2_PLACEMENT_3D('',#8617,#6757,#6758);
#5952=AXIS2_PLACEMENT_3D('',#8619,#6759,#6760);
#5953=AXIS2_PLACEMENT_3D('',#8622,#6762,#6763);
#5954=AXIS2_PLACEMENT_3D('',#8623,#6764,#6765);
#5955=AXIS2_PLACEMENT_3D('',#8624,#6766,#6767);
#5956=AXIS2_PLACEMENT_3D('',#8626,#6768,#6769);
#5957=AXIS2_PLACEMENT_3D('',#8629,#6771,#6772);
#5958=AXIS2_PLACEMENT_3D('',#8630,#6773,#6774);
#5959=AXIS2_PLACEMENT_3D('',#8631,#6775,#6776);
#5960=AXIS2_PLACEMENT_3D('',#8633,#6777,#6778);
#5961=AXIS2_PLACEMENT_3D('',#8636,#6780,#6781);
#5962=AXIS2_PLACEMENT_3D('',#8637,#6782,#6783);
#5963=AXIS2_PLACEMENT_3D('',#8638,#6784,#6785);
#5964=AXIS2_PLACEMENT_3D('',#8640,#6786,#6787);
#5965=AXIS2_PLACEMENT_3D('',#8643,#6789,#6790);
#5966=AXIS2_PLACEMENT_3D('',#8644,#6791,#6792);
#5967=AXIS2_PLACEMENT_3D('',#8645,#6793,#6794);
#5968=AXIS2_PLACEMENT_3D('',#8647,#6795,#6796);
#5969=AXIS2_PLACEMENT_3D('',#8650,#6798,#6799);
#5970=AXIS2_PLACEMENT_3D('',#8651,#6800,#6801);
#5971=AXIS2_PLACEMENT_3D('',#8652,#6802,#6803);
#5972=AXIS2_PLACEMENT_3D('',#8654,#6804,#6805);
#5973=AXIS2_PLACEMENT_3D('',#8657,#6807,#6808);
#5974=AXIS2_PLACEMENT_3D('',#8658,#6809,#6810);
#5975=AXIS2_PLACEMENT_3D('',#8659,#6811,#6812);
#5976=AXIS2_PLACEMENT_3D('',#8661,#6813,#6814);
#5977=AXIS2_PLACEMENT_3D('',#8664,#6816,#6817);
#5978=AXIS2_PLACEMENT_3D('',#8665,#6818,#6819);
#5979=AXIS2_PLACEMENT_3D('',#8666,#6820,#6821);
#5980=AXIS2_PLACEMENT_3D('',#8668,#6822,#6823);
#5981=AXIS2_PLACEMENT_3D('',#8671,#6825,#6826);
#5982=AXIS2_PLACEMENT_3D('',#8672,#6827,#6828);
#5983=AXIS2_PLACEMENT_3D('',#8674,#6829,#6830);
#5984=AXIS2_PLACEMENT_3D('',#8677,#6832,#6833);
#5985=AXIS2_PLACEMENT_3D('',#8678,#6834,#6835);
#5986=AXIS2_PLACEMENT_3D('',#8680,#6836,#6837);
#5987=AXIS2_PLACEMENT_3D('',#8683,#6839,#6840);
#5988=AXIS2_PLACEMENT_3D('',#8684,#6841,#6842);
#5989=AXIS2_PLACEMENT_3D('',#8686,#6843,#6844);
#5990=AXIS2_PLACEMENT_3D('',#8689,#6846,#6847);
#5991=AXIS2_PLACEMENT_3D('',#8690,#6848,#6849);
#5992=AXIS2_PLACEMENT_3D('',#8693,#6850,#6851);
#5993=AXIS2_PLACEMENT_3D('',#8699,#6855,#6856);
#5994=AXIS2_PLACEMENT_3D('',#8701,#6857,#6858);
#5995=AXIS2_PLACEMENT_3D('',#8707,#6862,#6863);
#5996=AXIS2_PLACEMENT_3D('',#8710,#6864,#6865);
#5997=AXIS2_PLACEMENT_3D('',#8716,#6869,#6870);
#5998=AXIS2_PLACEMENT_3D('',#8718,#6871,#6872);
#5999=AXIS2_PLACEMENT_3D('',#8724,#6876,#6877);
#6000=AXIS2_PLACEMENT_3D('',#8727,#6880,#6881);
#6001=AXIS2_PLACEMENT_3D('',#8730,#6884,#6885);
#6002=AXIS2_PLACEMENT_3D('',#8732,#6887,#6888);
#6003=AXIS2_PLACEMENT_3D('',#8734,#6890,#6891);
#6004=AXIS2_PLACEMENT_3D('',#8735,#6892,#6893);
#6005=AXIS2_PLACEMENT_3D('',#8738,#6894,#6895);
#6006=AXIS2_PLACEMENT_3D('',#8744,#6899,#6900);
#6007=AXIS2_PLACEMENT_3D('',#8746,#6901,#6902);
#6008=AXIS2_PLACEMENT_3D('',#8752,#6906,#6907);
#6009=AXIS2_PLACEMENT_3D('',#8755,#6908,#6909);
#6010=AXIS2_PLACEMENT_3D('',#8761,#6913,#6914);
#6011=AXIS2_PLACEMENT_3D('',#8763,#6915,#6916);
#6012=AXIS2_PLACEMENT_3D('',#8769,#6920,#6921);
#6013=AXIS2_PLACEMENT_3D('',#8772,#6924,#6925);
#6014=AXIS2_PLACEMENT_3D('',#8775,#6928,#6929);
#6015=AXIS2_PLACEMENT_3D('',#8777,#6931,#6932);
#6016=AXIS2_PLACEMENT_3D('',#8779,#6934,#6935);
#6017=AXIS2_PLACEMENT_3D('',#8780,#6936,#6937);
#6018=AXIS2_PLACEMENT_3D('',#8782,#6938,#6939);
#6019=AXIS2_PLACEMENT_3D('',#8785,#6941,#6942);
#6020=AXIS2_PLACEMENT_3D('',#8786,#6943,#6944);
#6021=AXIS2_PLACEMENT_3D('',#8788,#6945,#6946);
#6022=AXIS2_PLACEMENT_3D('',#8791,#6948,#6949);
#6023=AXIS2_PLACEMENT_3D('',#8792,#6950,#6951);
#6024=AXIS2_PLACEMENT_3D('',#8793,#6952,#6953);
#6746=DIRECTION('axis',(0.,0.,1.));
#6747=DIRECTION('refdir',(1.,0.,0.));
#6748=DIRECTION('center_axis',(0.,1.,0.));
#6749=DIRECTION('ref_axis',(1.,0.,0.));
#6750=DIRECTION('center_axis',(0.,1.,0.));
#6751=DIRECTION('ref_axis',(1.,0.,0.));
#6752=DIRECTION('',(0.,1.,0.));
#6753=DIRECTION('center_axis',(0.,-1.,0.));
#6754=DIRECTION('ref_axis',(1.,0.,0.));
#6755=DIRECTION('center_axis',(0.,1.,0.));
#6756=DIRECTION('ref_axis',(1.,0.,0.));
#6757=DIRECTION('center_axis',(0.,1.,0.));
#6758=DIRECTION('ref_axis',(1.,0.,0.));
#6759=DIRECTION('center_axis',(0.,1.,0.));
#6760=DIRECTION('ref_axis',(1.,0.,0.));
#6761=DIRECTION('',(0.,1.,0.));
#6762=DIRECTION('center_axis',(0.,-1.,0.));
#6763=DIRECTION('ref_axis',(1.,0.,0.));
#6764=DIRECTION('center_axis',(0.,1.,0.));
#6765=DIRECTION('ref_axis',(1.,0.,0.));
#6766=DIRECTION('center_axis',(0.,1.,0.));
#6767=DIRECTION('ref_axis',(1.,0.,0.));
#6768=DIRECTION('center_axis',(0.,1.,0.));
#6769=DIRECTION('ref_axis',(1.,0.,0.));
#6770=DIRECTION('',(0.,1.,0.));
#6771=DIRECTION('center_axis',(0.,-1.,0.));
#6772=DIRECTION('ref_axis',(1.,0.,0.));
#6773=DIRECTION('center_axis',(0.,1.,0.));
#6774=DIRECTION('ref_axis',(1.,0.,0.));
#6775=DIRECTION('center_axis',(0.,1.,0.));
#6776=DIRECTION('ref_axis',(1.,0.,0.));
#6777=DIRECTION('center_axis',(0.,1.,0.));
#6778=DIRECTION('ref_axis',(1.,0.,0.));
#6779=DIRECTION('',(0.,1.,0.));
#6780=DIRECTION('center_axis',(0.,-1.,0.));
#6781=DIRECTION('ref_axis',(1.,0.,0.));
#6782=DIRECTION('center_axis',(0.,1.,0.));
#6783=DIRECTION('ref_axis',(1.,0.,0.));
#6784=DIRECTION('center_axis',(0.,1.,0.));
#6785=DIRECTION('ref_axis',(1.,0.,0.));
#6786=DIRECTION('center_axis',(0.,1.,0.));
#6787=DIRECTION('ref_axis',(1.,0.,0.));
#6788=DIRECTION('',(0.,1.,0.));
#6789=DIRECTION('center_axis',(0.,1.,0.));
#6790=DIRECTION('ref_axis',(1.,0.,0.));
#6791=DIRECTION('center_axis',(0.,1.,0.));
#6792=DIRECTION('ref_axis',(1.,0.,0.));
#6793=DIRECTION('center_axis',(0.,1.,0.));
#6794=DIRECTION('ref_axis',(1.,0.,0.));
#6795=DIRECTION('center_axis',(0.,1.,0.));
#6796=DIRECTION('ref_axis',(1.,0.,0.));
#6797=DIRECTION('',(0.,1.,0.));
#6798=DIRECTION('center_axis',(0.,1.,0.));
#6799=DIRECTION('ref_axis',(1.,0.,0.));
#6800=DIRECTION('center_axis',(0.,1.,0.));
#6801=DIRECTION('ref_axis',(1.,0.,0.));
#6802=DIRECTION('center_axis',(0.,1.,0.));
#6803=DIRECTION('ref_axis',(1.,0.,0.));
#6804=DIRECTION('center_axis',(0.,1.,0.));
#6805=DIRECTION('ref_axis',(1.,0.,0.));
#6806=DIRECTION('',(0.,1.,0.));
#6807=DIRECTION('center_axis',(0.,1.,0.));
#6808=DIRECTION('ref_axis',(1.,0.,0.));
#6809=DIRECTION('center_axis',(0.,1.,0.));
#6810=DIRECTION('ref_axis',(1.,0.,0.));
#6811=DIRECTION('center_axis',(0.,1.,0.));
#6812=DIRECTION('ref_axis',(1.,0.,0.));
#6813=DIRECTION('center_axis',(0.,1.,0.));
#6814=DIRECTION('ref_axis',(1.,0.,0.));
#6815=DIRECTION('',(0.,1.,0.));
#6816=DIRECTION('center_axis',(0.,1.,0.));
#6817=DIRECTION('ref_axis',(1.,0.,0.));
#6818=DIRECTION('center_axis',(0.,1.,0.));
#6819=DIRECTION('ref_axis',(1.,0.,0.));
#6820=DIRECTION('center_axis',(0.,0.,1.));
#6821=DIRECTION('ref_axis',(1.,0.,0.));
#6822=DIRECTION('center_axis',(0.,0.,1.));
#6823=DIRECTION('ref_axis',(1.,0.,0.));
#6824=DIRECTION('',(0.,0.,1.));
#6825=DIRECTION('center_axis',(0.,0.,-1.));
#6826=DIRECTION('ref_axis',(1.,0.,0.));
#6827=DIRECTION('center_axis',(0.,0.,1.));
#6828=DIRECTION('ref_axis',(1.,0.,0.));
#6829=DIRECTION('center_axis',(0.,0.,1.));
#6830=DIRECTION('ref_axis',(1.,0.,0.));
#6831=DIRECTION('',(0.,0.,1.));
#6832=DIRECTION('center_axis',(0.,0.,-1.));
#6833=DIRECTION('ref_axis',(1.,0.,0.));
#6834=DIRECTION('center_axis',(0.,0.,1.));
#6835=DIRECTION('ref_axis',(1.,0.,0.));
#6836=DIRECTION('center_axis',(0.,0.,1.));
#6837=DIRECTION('ref_axis',(1.,0.,0.));
#6838=DIRECTION('',(0.,0.,1.));
#6839=DIRECTION('center_axis',(0.,0.,-1.));
#6840=DIRECTION('ref_axis',(1.,0.,0.));
#6841=DIRECTION('center_axis',(0.,0.,1.));
#6842=DIRECTION('ref_axis',(1.,0.,0.));
#6843=DIRECTION('center_axis',(0.,0.,1.));
#6844=DIRECTION('ref_axis',(1.,0.,0.));
#6845=DIRECTION('',(0.,0.,1.));
#6846=DIRECTION('center_axis',(0.,0.,-1.));
#6847=DIRECTION('ref_axis',(1.,0.,0.));
#6848=DIRECTION('center_axis',(0.,1.,0.));
#6849=DIRECTION('ref_axis',(0.,0.,1.));
#6850=DIRECTION('center_axis',(0.,1.,0.));
#6851=DIRECTION('ref_axis',(1.,0.,0.));
#6852=DIRECTION('',(1.,0.,0.));
#6853=DIRECTION('',(0.,0.,-1.));
#6854=DIRECTION('',(-1.,0.,0.));
#6855=DIRECTION('center_axis',(0.,1.,0.));
#6856=DIRECTION('ref_axis',(0.,0.,1.));
#6857=DIRECTION('center_axis',(0.,1.,0.));
#6858=DIRECTION('ref_axis',(1.,0.,0.));
#6859=DIRECTION('',(-1.,0.,0.));
#6860=DIRECTION('',(0.,0.,1.));
#6861=DIRECTION('',(1.,0.,0.));
#6862=DIRECTION('center_axis',(0.,1.,0.));
#6863=DIRECTION('ref_axis',(1.,0.,0.));
#6864=DIRECTION('center_axis',(0.,-1.,0.));
#6865=DIRECTION('ref_axis',(1.,0.,0.));
#6866=DIRECTION('',(1.,0.,0.));
#6867=DIRECTION('',(0.,0.,1.));
#6868=DIRECTION('',(-1.,0.,0.));
#6869=DIRECTION('center_axis',(0.,1.,0.));
#6870=DIRECTION('ref_axis',(1.,0.,0.));
#6871=DIRECTION('center_axis',(0.,-1.,0.));
#6872=DIRECTION('ref_axis',(1.,0.,0.));
#6873=DIRECTION('',(-1.,0.,0.));
#6874=DIRECTION('',(0.,0.,-1.));
#6875=DIRECTION('',(1.,0.,0.));
#6876=DIRECTION('center_axis',(0.,0.,1.));
#6877=DIRECTION('ref_axis',(1.,0.,0.));
#6878=DIRECTION('',(0.,1.,0.));
#6879=DIRECTION('',(0.,1.,0.));
#6880=DIRECTION('center_axis',(0.,0.,1.));
#6881=DIRECTION('ref_axis',(1.,0.,0.));
#6882=DIRECTION('',(0.,-1.,0.));
#6883=DIRECTION('',(0.,1.,0.));
#6884=DIRECTION('center_axis',(-1.,0.,0.));
#6885=DIRECTION('ref_axis',(0.,0.,1.));
#6886=DIRECTION('',(0.,1.,0.));
#6887=DIRECTION('center_axis',(0.,0.,-1.));
#6888=DIRECTION('ref_axis',(-1.,0.,0.));
#6889=DIRECTION('',(0.,1.,0.));
#6890=DIRECTION('center_axis',(1.,0.,0.));
#6891=DIRECTION('ref_axis',(0.,0.,-1.));
#6892=DIRECTION('center_axis',(0.,1.,0.));
#6893=DIRECTION('ref_axis',(0.,0.,1.));
#6894=DIRECTION('center_axis',(0.,1.,0.));
#6895=DIRECTION('ref_axis',(1.,0.,0.));
#6896=DIRECTION('',(1.,0.,0.));
#6897=DIRECTION('',(0.,0.,-1.));
#6898=DIRECTION('',(-1.,0.,0.));
#6899=DIRECTION('center_axis',(0.,1.,0.));
#6900=DIRECTION('ref_axis',(0.,0.,1.));
#6901=DIRECTION('center_axis',(0.,1.,0.));
#6902=DIRECTION('ref_axis',(1.,0.,0.));
#6903=DIRECTION('',(-1.,0.,0.));
#6904=DIRECTION('',(0.,0.,1.));
#6905=DIRECTION('',(1.,0.,0.));
#6906=DIRECTION('center_axis',(0.,1.,0.));
#6907=DIRECTION('ref_axis',(1.,0.,0.));
#6908=DIRECTION('center_axis',(0.,-1.,0.));
#6909=DIRECTION('ref_axis',(1.,0.,0.));
#6910=DIRECTION('',(1.,0.,0.));
#6911=DIRECTION('',(0.,0.,1.));
#6912=DIRECTION('',(-1.,0.,0.));
#6913=DIRECTION('center_axis',(0.,1.,0.));
#6914=DIRECTION('ref_axis',(1.,0.,0.));
#6915=DIRECTION('center_axis',(0.,-1.,0.));
#6916=DIRECTION('ref_axis',(1.,0.,0.));
#6917=DIRECTION('',(-1.,0.,0.));
#6918=DIRECTION('',(0.,0.,-1.));
#6919=DIRECTION('',(1.,0.,0.));
#6920=DIRECTION('center_axis',(0.,0.,1.));
#6921=DIRECTION('ref_axis',(1.,0.,0.));
#6922=DIRECTION('',(0.,1.,0.));
#6923=DIRECTION('',(0.,1.,0.));
#6924=DIRECTION('center_axis',(0.,0.,1.));
#6925=DIRECTION('ref_axis',(1.,0.,0.));
#6926=DIRECTION('',(0.,-1.,0.));
#6927=DIRECTION('',(0.,1.,0.));
#6928=DIRECTION('center_axis',(-1.,0.,0.));
#6929=DIRECTION('ref_axis',(0.,0.,1.));
#6930=DIRECTION('',(0.,1.,0.));
#6931=DIRECTION('center_axis',(0.,0.,-1.));
#6932=DIRECTION('ref_axis',(-1.,0.,0.));
#6933=DIRECTION('',(0.,1.,0.));
#6934=DIRECTION('center_axis',(1.,0.,0.));
#6935=DIRECTION('ref_axis',(0.,0.,-1.));
#6936=DIRECTION('center_axis',(0.,1.,0.));
#6937=DIRECTION('ref_axis',(1.,0.,0.));
#6938=DIRECTION('center_axis',(0.,-1.,0.));
#6939=DIRECTION('ref_axis',(1.,0.,0.));
#6940=DIRECTION('',(0.,-1.,0.));
#6941=DIRECTION('center_axis',(0.,-1.,0.));
#6942=DIRECTION('ref_axis',(1.,0.,0.));
#6943=DIRECTION('center_axis',(0.,1.,0.));
#6944=DIRECTION('ref_axis',(1.,0.,0.));
#6945=DIRECTION('center_axis',(0.,1.,0.));
#6946=DIRECTION('ref_axis',(1.,0.,0.));
#6947=DIRECTION('',(0.,-1.,0.));
#6948=DIRECTION('center_axis',(0.,1.,0.));
#6949=DIRECTION('ref_axis',(1.,0.,0.));
#6950=DIRECTION('center_axis',(0.,1.,0.));
#6951=DIRECTION('ref_axis',(1.,0.,0.));
#6952=DIRECTION('center_axis',(0.,1.,0.));
#6953=DIRECTION('ref_axis',(1.,0.,0.));
#8609=CARTESIAN_POINT('',(0.,0.,0.));
#8610=CARTESIAN_POINT('Origin',(-2.8,4.4,4.5));
#8611=CARTESIAN_POINT('',(-2.965,4.4,4.5));
#8612=CARTESIAN_POINT('Origin',(-2.8,4.4,4.5));
#8613=CARTESIAN_POINT('',(-2.965,6.,4.5));
#8614=CARTESIAN_POINT('',(-2.965,4.4,4.5));
#8615=CARTESIAN_POINT('Origin',(-2.8,6.,4.5));
#8616=CARTESIAN_POINT('Origin',(-2.8,4.4,4.5));
#8617=CARTESIAN_POINT('Origin',(1.71450551880629E-16,4.4,7.3));
#8618=CARTESIAN_POINT('',(-0.165,4.4,7.3));
#8619=CARTESIAN_POINT('Origin',(1.71450551880629E-16,4.4,7.3));
#8620=CARTESIAN_POINT('',(-0.165,6.,7.3));
#8621=CARTESIAN_POINT('',(-0.165,4.4,7.3));
#8622=CARTESIAN_POINT('Origin',(1.71450551880629E-16,6.,7.3));
#8623=CARTESIAN_POINT('Origin',(1.66533453693773E-16,4.4,7.3));
#8624=CARTESIAN_POINT('Origin',(2.8,4.4,4.5));
#8625=CARTESIAN_POINT('',(2.635,4.4,4.5));
#8626=CARTESIAN_POINT('Origin',(2.8,4.4,4.5));
#8627=CARTESIAN_POINT('',(2.635,6.,4.5));
#8628=CARTESIAN_POINT('',(2.635,4.4,4.5));
#8629=CARTESIAN_POINT('Origin',(2.8,6.,4.5));
#8630=CARTESIAN_POINT('Origin',(2.8,4.4,4.5));
#8631=CARTESIAN_POINT('Origin',(-5.14351655641888E-16,4.4,1.7));
#8632=CARTESIAN_POINT('',(-0.165000000000001,4.4,1.7));
#8633=CARTESIAN_POINT('Origin',(-5.14351655641888E-16,4.4,1.7));
#8634=CARTESIAN_POINT('',(-0.165000000000001,6.,1.7));
#8635=CARTESIAN_POINT('',(-0.165000000000001,4.4,1.7));
#8636=CARTESIAN_POINT('Origin',(-5.14351655641888E-16,6.,1.7));
#8637=CARTESIAN_POINT('Origin',(-5.27355936696949E-16,4.4,1.7));
#8638=CARTESIAN_POINT('Origin',(-2.8,-0.1,4.5));
#8639=CARTESIAN_POINT('',(-2.965,0.,4.5));
#8640=CARTESIAN_POINT('Origin',(-2.8,0.,4.5));
#8641=CARTESIAN_POINT('',(-2.965,1.6,4.5));
#8642=CARTESIAN_POINT('',(-2.965,-0.1,4.5));
#8643=CARTESIAN_POINT('Origin',(-2.8,1.6,4.5));
#8644=CARTESIAN_POINT('Origin',(-2.8,1.6,4.5));
#8645=CARTESIAN_POINT('Origin',(1.71450551880629E-16,-0.1,7.3));
#8646=CARTESIAN_POINT('',(-0.165,0.,7.3));
#8647=CARTESIAN_POINT('Origin',(1.71450551880629E-16,0.,7.3));
#8648=CARTESIAN_POINT('',(-0.165,1.6,7.3));
#8649=CARTESIAN_POINT('',(-0.165,-0.1,7.3));
#8650=CARTESIAN_POINT('Origin',(1.71450551880629E-16,1.6,7.3));
#8651=CARTESIAN_POINT('Origin',(1.66533453693773E-16,1.6,7.3));
#8652=CARTESIAN_POINT('Origin',(2.8,-0.1,4.5));
#8653=CARTESIAN_POINT('',(2.635,0.,4.5));
#8654=CARTESIAN_POINT('Origin',(2.8,0.,4.5));
#8655=CARTESIAN_POINT('',(2.635,1.6,4.5));
#8656=CARTESIAN_POINT('',(2.635,-0.1,4.5));
#8657=CARTESIAN_POINT('Origin',(2.8,1.6,4.5));
#8658=CARTESIAN_POINT('Origin',(2.8,1.6,4.5));
#8659=CARTESIAN_POINT('Origin',(-5.14351655641888E-16,-0.1,1.7));
#8660=CARTESIAN_POINT('',(-0.165000000000001,0.,1.7));
#8661=CARTESIAN_POINT('Origin',(-5.14351655641888E-16,0.,1.7));
#8662=CARTESIAN_POINT('',(-0.165000000000001,1.6,1.7));
#8663=CARTESIAN_POINT('',(-0.165000000000001,-0.1,1.7));
#8664=CARTESIAN_POINT('Origin',(-5.14351655641888E-16,1.6,1.7));
#8665=CARTESIAN_POINT('Origin',(-5.27355936696949E-16,1.6,1.7));
#8666=CARTESIAN_POINT('Origin',(3.8,1.,0.9));
#8667=CARTESIAN_POINT('',(3.47,1.,1.));
#8668=CARTESIAN_POINT('Origin',(3.8,1.,1.));
#8669=CARTESIAN_POINT('',(3.47,1.,2.5));
#8670=CARTESIAN_POINT('',(3.47,1.,0.9));
#8671=CARTESIAN_POINT('Origin',(3.8,1.,2.5));
#8672=CARTESIAN_POINT('Origin',(-3.8,5.,0.9));
#8673=CARTESIAN_POINT('',(-4.13,5.,1.));
#8674=CARTESIAN_POINT('Origin',(-3.8,5.,1.));
#8675=CARTESIAN_POINT('',(-4.13,5.,2.5));
#8676=CARTESIAN_POINT('',(-4.13,5.,0.9));
#8677=CARTESIAN_POINT('Origin',(-3.8,5.,2.5));
#8678=CARTESIAN_POINT('Origin',(-3.8,1.,0.9));
#8679=CARTESIAN_POINT('',(-4.13,1.,1.));
#8680=CARTESIAN_POINT('Origin',(-3.8,1.,1.));
#8681=CARTESIAN_POINT('',(-4.13,1.,2.5));
#8682=CARTESIAN_POINT('',(-4.13,1.,0.9));
#8683=CARTESIAN_POINT('Origin',(-3.8,1.,2.5));
#8684=CARTESIAN_POINT('Origin',(3.8,5.,0.9));
#8685=CARTESIAN_POINT('',(3.47,5.,1.));
#8686=CARTESIAN_POINT('Origin',(3.8,5.,1.));
#8687=CARTESIAN_POINT('',(3.47,5.,2.5));
#8688=CARTESIAN_POINT('',(3.47,5.,0.9));
#8689=CARTESIAN_POINT('Origin',(3.8,5.,2.5));
#8690=CARTESIAN_POINT('Origin',(0.,5.5,1.75));
#8691=CARTESIAN_POINT('',(2.87228132326901,5.5,2.5));
#8692=CARTESIAN_POINT('',(0.,5.5,1.));
#8693=CARTESIAN_POINT('Origin',(0.,5.5,4.5));
#8694=CARTESIAN_POINT('',(4.5,5.5,2.5));
#8695=CARTESIAN_POINT('',(4.5,5.5,2.5));
#8696=CARTESIAN_POINT('',(4.5,5.5,1.));
#8697=CARTESIAN_POINT('',(4.5,5.5,1.));
#8698=CARTESIAN_POINT('',(-4.5,5.5,1.));
#8699=CARTESIAN_POINT('Origin',(0.,5.5,1.75));
#8700=CARTESIAN_POINT('',(-2.87228132326901,5.5,2.5));
#8701=CARTESIAN_POINT('Origin',(0.,5.5,4.5));
#8702=CARTESIAN_POINT('',(-4.5,5.5,1.));
#8703=CARTESIAN_POINT('',(-4.5,5.5,1.));
#8704=CARTESIAN_POINT('',(-4.5,5.5,2.5));
#8705=CARTESIAN_POINT('',(-4.5,5.5,2.5));
#8706=CARTESIAN_POINT('',(4.5,5.5,2.5));
#8707=CARTESIAN_POINT('Origin',(0.,4.5,1.75));
#8708=CARTESIAN_POINT('',(0.,4.5,1.));
#8709=CARTESIAN_POINT('',(2.87228132326901,4.5,2.5));
#8710=CARTESIAN_POINT('Origin',(0.,4.5,4.5));
#8711=CARTESIAN_POINT('',(4.5,4.5,1.));
#8712=CARTESIAN_POINT('',(-4.5,4.5,1.));
#8713=CARTESIAN_POINT('',(4.5,4.5,2.5));
#8714=CARTESIAN_POINT('',(4.5,4.5,1.));
#8715=CARTESIAN_POINT('',(4.5,4.5,2.5));
#8716=CARTESIAN_POINT('Origin',(0.,4.5,1.75));
#8717=CARTESIAN_POINT('',(-2.87228132326901,4.5,2.5));
#8718=CARTESIAN_POINT('Origin',(0.,4.5,4.5));
#8719=CARTESIAN_POINT('',(-4.5,4.5,2.5));
#8720=CARTESIAN_POINT('',(4.5,4.5,2.5));
#8721=CARTESIAN_POINT('',(-4.5,4.5,1.));
#8722=CARTESIAN_POINT('',(-4.5,4.5,2.5));
#8723=CARTESIAN_POINT('',(-4.5,4.5,1.));
#8724=CARTESIAN_POINT('Origin',(-4.5,4.5,2.5));
#8725=CARTESIAN_POINT('',(2.87228132326901,0.,2.5));
#8726=CARTESIAN_POINT('',(4.5,4.5,2.5));
#8727=CARTESIAN_POINT('Origin',(-4.5,4.5,2.5));
#8728=CARTESIAN_POINT('',(-2.87228132326901,0.,2.5));
#8729=CARTESIAN_POINT('',(-4.5,4.5,2.5));
#8730=CARTESIAN_POINT('Origin',(-4.5,4.5,1.));
#8731=CARTESIAN_POINT('',(-4.5,4.5,1.));
#8732=CARTESIAN_POINT('Origin',(4.5,4.5,1.));
#8733=CARTESIAN_POINT('',(4.5,4.5,1.));
#8734=CARTESIAN_POINT('Origin',(4.5,4.5,2.5));
#8735=CARTESIAN_POINT('Origin',(0.,1.5,1.75));
#8736=CARTESIAN_POINT('',(2.87228132326901,1.5,2.5));
#8737=CARTESIAN_POINT('',(0.,1.5,1.));
#8738=CARTESIAN_POINT('Origin',(0.,1.5,4.5));
#8739=CARTESIAN_POINT('',(4.5,1.5,2.5));
#8740=CARTESIAN_POINT('',(4.5,1.5,2.5));
#8741=CARTESIAN_POINT('',(4.5,1.5,1.));
#8742=CARTESIAN_POINT('',(4.5,1.5,1.));
#8743=CARTESIAN_POINT('',(-4.5,1.5,1.));
#8744=CARTESIAN_POINT('Origin',(0.,1.5,1.75));
#8745=CARTESIAN_POINT('',(-2.87228132326901,1.5,2.5));
#8746=CARTESIAN_POINT('Origin',(0.,1.5,4.5));
#8747=CARTESIAN_POINT('',(-4.5,1.5,1.));
#8748=CARTESIAN_POINT('',(-4.5,1.5,1.));
#8749=CARTESIAN_POINT('',(-4.5,1.5,2.5));
#8750=CARTESIAN_POINT('',(-4.5,1.5,2.5));
#8751=CARTESIAN_POINT('',(4.5,1.5,2.5));
#8752=CARTESIAN_POINT('Origin',(0.,0.5,1.75));
#8753=CARTESIAN_POINT('',(0.,0.5,1.));
#8754=CARTESIAN_POINT('',(2.87228132326901,0.5,2.5));
#8755=CARTESIAN_POINT('Origin',(0.,0.5,4.5));
#8756=CARTESIAN_POINT('',(4.5,0.5,1.));
#8757=CARTESIAN_POINT('',(-4.5,0.5,1.));
#8758=CARTESIAN_POINT('',(4.5,0.5,2.5));
#8759=CARTESIAN_POINT('',(4.5,0.5,1.));
#8760=CARTESIAN_POINT('',(4.5,0.5,2.5));
#8761=CARTESIAN_POINT('Origin',(0.,0.5,1.75));
#8762=CARTESIAN_POINT('',(-2.87228132326901,0.5,2.5));
#8763=CARTESIAN_POINT('Origin',(0.,0.5,4.5));
#8764=CARTESIAN_POINT('',(-4.5,0.5,2.5));
#8765=CARTESIAN_POINT('',(4.5,0.5,2.5));
#8766=CARTESIAN_POINT('',(-4.5,0.5,1.));
#8767=CARTESIAN_POINT('',(-4.5,0.5,2.5));
#8768=CARTESIAN_POINT('',(-4.5,0.5,1.));
#8769=CARTESIAN_POINT('Origin',(-4.5,0.5,2.5));
#8770=CARTESIAN_POINT('',(2.87228132326901,0.,2.5));
#8771=CARTESIAN_POINT('',(4.5,0.5,2.5));
#8772=CARTESIAN_POINT('Origin',(-4.5,0.5,2.5));
#8773=CARTESIAN_POINT('',(-2.87228132326901,0.,2.5));
#8774=CARTESIAN_POINT('',(-4.5,0.5,2.5));
#8775=CARTESIAN_POINT('Origin',(-4.5,0.5,1.));
#8776=CARTESIAN_POINT('',(-4.5,0.5,1.));
#8777=CARTESIAN_POINT('Origin',(4.5,0.5,1.));
#8778=CARTESIAN_POINT('',(4.5,0.5,1.));
#8779=CARTESIAN_POINT('Origin',(4.5,0.5,2.5));
#8780=CARTESIAN_POINT('Origin',(0.,0.,4.5));
#8781=CARTESIAN_POINT('',(-2.35,6.,4.5));
#8782=CARTESIAN_POINT('Origin',(0.,6.,4.5));
#8783=CARTESIAN_POINT('',(-2.35,0.,4.5));
#8784=CARTESIAN_POINT('',(-2.35,0.,4.5));
#8785=CARTESIAN_POINT('Origin',(0.,0.,4.5));
#8786=CARTESIAN_POINT('Origin',(0.,0.,4.5));
#8787=CARTESIAN_POINT('',(-3.5,6.,4.5));
#8788=CARTESIAN_POINT('Origin',(0.,6.,4.5));
#8789=CARTESIAN_POINT('',(-3.5,0.,4.5));
#8790=CARTESIAN_POINT('',(-3.5,0.,4.5));
#8791=CARTESIAN_POINT('Origin',(0.,0.,4.5));
#8792=CARTESIAN_POINT('Origin',(0.,6.,4.5));
#8793=CARTESIAN_POINT('Origin',(0.,0.,4.5));
#10913=UNCERTAINTY_MEASURE_WITH_UNIT(LENGTH_MEASURE(0.001),#10964,
'DISTANCE_ACCURACY_VALUE',
'Maximum model space distance between geometric entities at asserted c
onnectivities');
#10936=UNCERTAINTY_MEASURE_WITH_UNIT(LENGTH_MEASURE(0.001),#10964,
'DISTANCE_ACCURACY_VALUE',
'Maximum model space distance between geometric entities at asserted c
onnectivities');
#10940=(
GEOMETRIC_REPRESENTATION_CONTEXT(3)
GLOBAL_UNCERTAINTY_ASSIGNED_CONTEXT((#10913))
GLOBAL_UNIT_ASSIGNED_CONTEXT((#10964,#10966,#10967))
REPRESENTATION_CONTEXT('','3D')
);
#10963=(
GEOMETRIC_REPRESENTATION_CONTEXT(3)
GLOBAL_UNCERTAINTY_ASSIGNED_CONTEXT((#10936))
GLOBAL_UNIT_ASSIGNED_CONTEXT((#10964,#10966,#10967))
REPRESENTATION_CONTEXT('','3D')
);
#10964=(
LENGTH_UNIT()
NAMED_UNIT(*)
SI_UNIT(.CENTI.,.METRE.)
);
#10966=(
NAMED_UNIT(*)
PLANE_ANGLE_UNIT()
SI_UNIT($,.RADIAN.)
);
#10967=(
NAMED_UNIT(*)
SI_UNIT($,.STERADIAN.)
SOLID_ANGLE_UNIT()
);
#10971=SHAPE_DEFINITION_REPRESENTATION(#10997,#11060);
#10997=PRODUCT_DEFINITION_SHAPE('',$,#11087);
#11060=SHAPE_REPRESENTATION('',(#5946),#10940);
#11083=PRODUCT_DEFINITION_CONTEXT('part definition',#11163,'design');
#11087=PRODUCT_DEFINITION('Housing','Housing',#11113,#11083);
#11113=PRODUCT_DEFINITION_FORMATION('',$,#11168);
#11163=APPLICATION_CONTEXT(
'Core Data for Automotive Mechanical Design Process');
#11164=PRODUCT_CONTEXT('part definition',#11163,'mechanical');
#11168=PRODUCT('Housing','Housing','Housing',(#11164));
#11226=COLOUR_RGB('Dark Blue',0.08,0.2,0.34);
#11227=FILL_AREA_STYLE_COLOUR('',#11226);
#11228=FILL_AREA_STYLE('',(#11227));
#11229=SURFACE_STYLE_FILL_AREA(#11228);
#11230=SURFACE_SIDE_STYLE('',(#11229));
#11231=SURFACE_STYLE_USAGE(.BOTH.,#11230);
#11232=PRESENTATION_STYLE_ASSIGNMENT((#11231));
ENDSEC;
END-ISO-10303-21;
